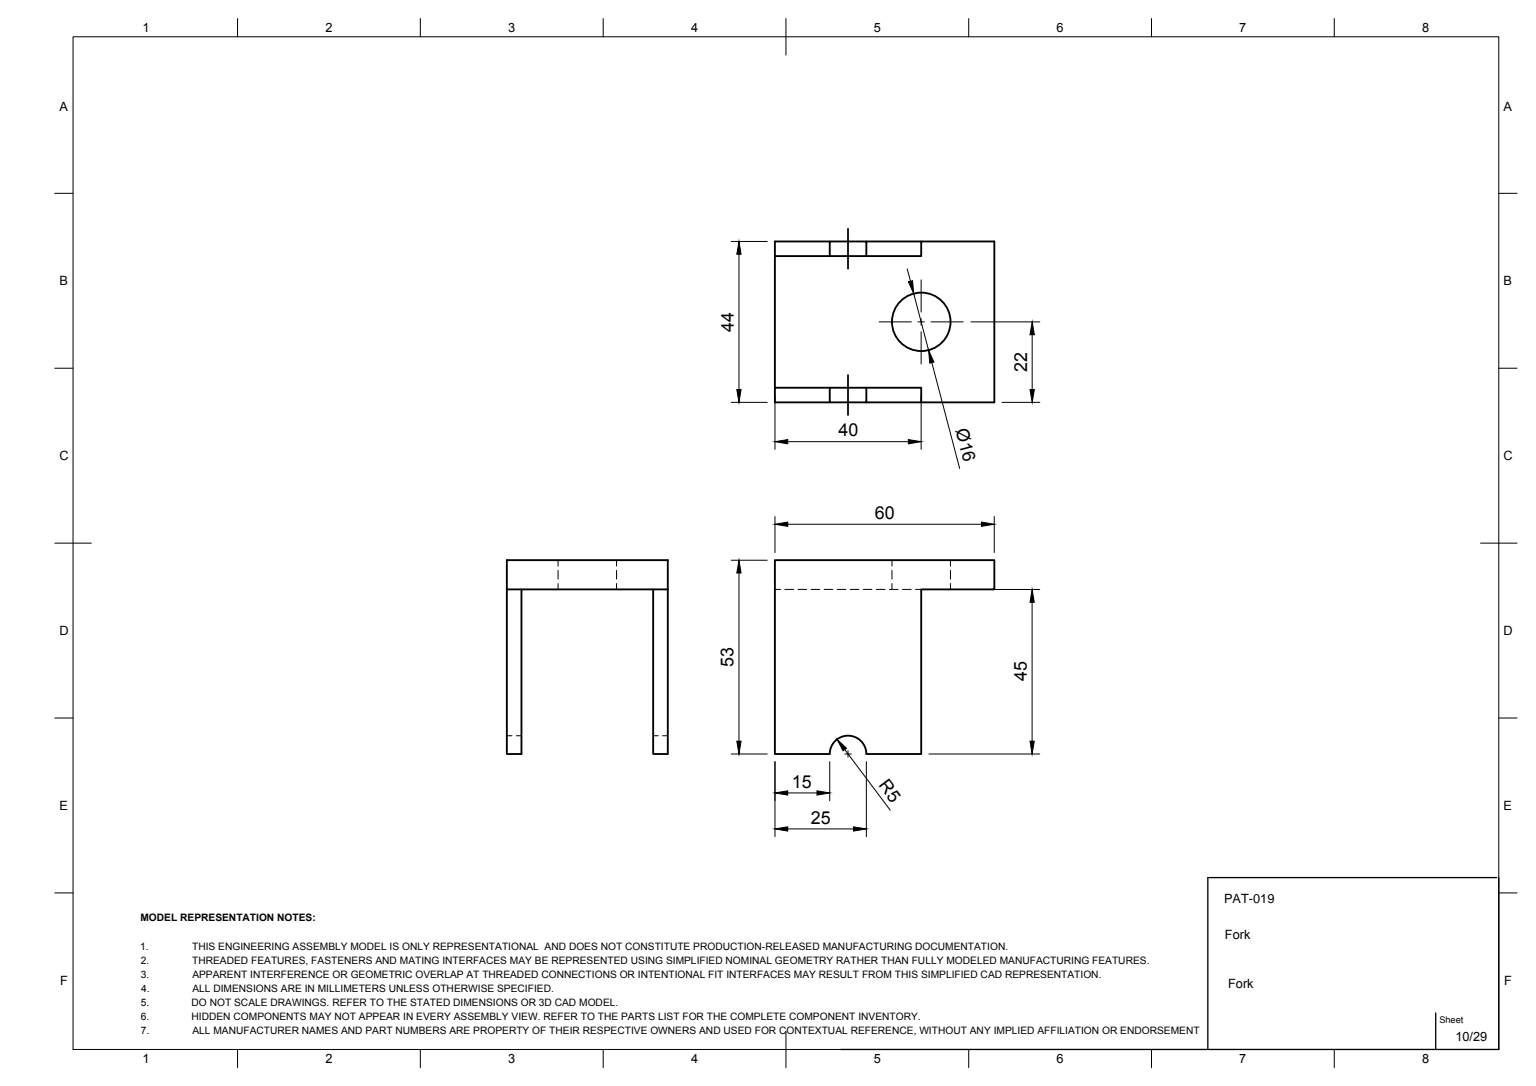
ISO-10303-21;
HEADER;
/* Generated by software containing ST-Developer
 * from STEP Tools, Inc. (www.steptools.com) 
 */

FILE_DESCRIPTION(
/* description */ ('Caster wheel assembly'),
/* implementation_level */ '2;1');

FILE_NAME(
/* name */ 'Fork.step',
/* time_stamp */ '2026-10-28T03:23:56-07:00',
/* author */ (''),
/* organization */ (''),
/* preprocessor_version */ 'ST-DEVELOPER v20.2',
/* originating_system */ 'Autodesk Translation Framework v15.17.0.0',
/* authorisation */ '');

FILE_SCHEMA (('AUTOMOTIVE_DESIGN { 1 0 10303 214 3 1 1 }'));
ENDSEC;

DATA;
#10=MECHANICAL_DESIGN_GEOMETRIC_PRESENTATION_REPRESENTATION('',(#227),#5385);
#183=SHAPE_REPRESENTATION_RELATIONSHIP('SRR','None',#5479,#205);
#205=ADVANCED_BREP_SHAPE_REPRESENTATION('',(#257),#5366);
#227=STYLED_ITEM('',(#5686),#257);
#257=MANIFOLD_SOLID_BREP('Body1',#2654);
#299=FACE_BOUND('',#655,.T.);
#300=FACE_BOUND('',#662,.T.);
#355=PLANE('',#3011);
#356=PLANE('',#3012);
#357=PLANE('',#3013);
#358=PLANE('',#3014);
#359=PLANE('',#3015);
#360=PLANE('',#3016);
#361=PLANE('',#3017);
#362=PLANE('',#3018);
#363=PLANE('',#3019);
#364=PLANE('',#3020);
#365=PLANE('',#3021);
#366=PLANE('',#3022);
#367=PLANE('',#3023);
#368=PLANE('',#3024);
#458=FACE_OUTER_BOUND('',#644,.T.);
#459=FACE_OUTER_BOUND('',#645,.T.);
#460=FACE_OUTER_BOUND('',#646,.T.);
#461=FACE_OUTER_BOUND('',#647,.T.);
#462=FACE_OUTER_BOUND('',#648,.T.);
#463=FACE_OUTER_BOUND('',#649,.T.);
#464=FACE_OUTER_BOUND('',#650,.T.);
#465=FACE_OUTER_BOUND('',#651,.T.);
#466=FACE_OUTER_BOUND('',#652,.T.);
#467=FACE_OUTER_BOUND('',#653,.T.);
#468=FACE_OUTER_BOUND('',#654,.T.);
#469=FACE_OUTER_BOUND('',#656,.T.);
#470=FACE_OUTER_BOUND('',#657,.T.);
#471=FACE_OUTER_BOUND('',#658,.T.);
#472=FACE_OUTER_BOUND('',#659,.T.);
#473=FACE_OUTER_BOUND('',#660,.T.);
#474=FACE_OUTER_BOUND('',#661,.T.);
#644=EDGE_LOOP('',(#1928,#1929,#1930,#1931));
#645=EDGE_LOOP('',(#1932,#1933,#1934,#1935));
#646=EDGE_LOOP('',(#1936,#1937,#1938,#1939));
#647=EDGE_LOOP('',(#1940,#1941,#1942,#1943,#1944,#1945,#1946,#1947));
#648=EDGE_LOOP('',(#1948,#1949,#1950,#1951));
#649=EDGE_LOOP('',(#1952,#1953,#1954,#1955));
#650=EDGE_LOOP('',(#1956,#1957,#1958,#1959,#1960,#1961,#1962,#1963));
#651=EDGE_LOOP('',(#1964,#1965,#1966,#1967));
#652=EDGE_LOOP('',(#1968,#1969,#1970,#1971));
#653=EDGE_LOOP('',(#1972,#1973,#1974,#1975,#1976,#1977));
#654=EDGE_LOOP('',(#1978,#1979,#1980,#1981,#1982,#1983,#1984,#1985));
#655=EDGE_LOOP('',(#1986));
#656=EDGE_LOOP('',(#1987,#1988,#1989,#1990,#1991,#1992,#1993,#1994));
#657=EDGE_LOOP('',(#1995,#1996,#1997,#1998,#1999,#2000));
#658=EDGE_LOOP('',(#2001,#2002,#2003,#2004));
#659=EDGE_LOOP('',(#2005,#2006,#2007,#2008));
#660=EDGE_LOOP('',(#2009,#2010,#2011,#2012));
#661=EDGE_LOOP('',(#2013,#2014,#2015,#2016));
#662=EDGE_LOOP('',(#2017));
#842=LINE('',#4400,#976);
#843=LINE('',#4407,#977);
#844=LINE('',#4410,#978);
#845=LINE('',#4414,#979);
#846=LINE('',#4418,#980);
#847=LINE('',#4422,#981);
#848=LINE('',#4424,#982);
#849=LINE('',#4426,#983);
#850=LINE('',#4428,#984);
#851=LINE('',#4430,#985);
#852=LINE('',#4432,#986);
#853=LINE('',#4433,#987);
#854=LINE('',#4436,#988);
#855=LINE('',#4437,#989);
#856=LINE('',#4440,#990);
#857=LINE('',#4441,#991);
#858=LINE('',#4444,#992);
#859=LINE('',#4446,#993);
#860=LINE('',#4448,#994);
#861=LINE('',#4450,#995);
#862=LINE('',#4452,#996);
#863=LINE('',#4454,#997);
#864=LINE('',#4455,#998);
#865=LINE('',#4458,#999);
#866=LINE('',#4459,#1000);
#867=LINE('',#4462,#1001);
#868=LINE('',#4463,#1002);
#869=LINE('',#4466,#1003);
#870=LINE('',#4467,#1004);
#871=LINE('',#4470,#1005);
#872=LINE('',#4472,#1006);
#873=LINE('',#4473,#1007);
#874=LINE('',#4474,#1008);
#875=LINE('',#4476,#1009);
#876=LINE('',#4477,#1010);
#877=LINE('',#4480,#1011);
#878=LINE('',#4481,#1012);
#879=LINE('',#4483,#1013);
#880=LINE('',#4486,#1014);
#976=VECTOR('',#3499,0.8);
#977=VECTOR('',#3506,1.);
#978=VECTOR('',#3509,1.);
#979=VECTOR('',#3512,1.);
#980=VECTOR('',#3515,1.);
#981=VECTOR('',#3520,1.);
#982=VECTOR('',#3521,1.);
#983=VECTOR('',#3522,1.);
#984=VECTOR('',#3523,1.);
#985=VECTOR('',#3524,1.);
#986=VECTOR('',#3525,1.);
#987=VECTOR('',#3526,1.);
#988=VECTOR('',#3529,1.);
#989=VECTOR('',#3530,1.);
#990=VECTOR('',#3533,1.);
#991=VECTOR('',#3534,1.);
#992=VECTOR('',#3537,1.);
#993=VECTOR('',#3538,1.);
#994=VECTOR('',#3539,1.);
#995=VECTOR('',#3540,1.);
#996=VECTOR('',#3541,1.);
#997=VECTOR('',#3542,1.);
#998=VECTOR('',#3543,1.);
#999=VECTOR('',#3546,1.);
#1000=VECTOR('',#3547,1.);
#1001=VECTOR('',#3550,1.);
#1002=VECTOR('',#3551,1.);
#1003=VECTOR('',#3554,1.);
#1004=VECTOR('',#3555,1.);
#1005=VECTOR('',#3558,1.);
#1006=VECTOR('',#3559,1.);
#1007=VECTOR('',#3560,1.);
#1008=VECTOR('',#3561,1.);
#1009=VECTOR('',#3564,1.);
#1010=VECTOR('',#3565,1.);
#1011=VECTOR('',#3568,1.);
#1012=VECTOR('',#3569,1.);
#1013=VECTOR('',#3572,1.);
#1014=VECTOR('',#3577,1.);
#1105=CIRCLE('',#3003,0.8);
#1106=CIRCLE('',#3004,0.8);
#1107=CIRCLE('',#3006,0.5);
#1108=CIRCLE('',#3007,0.5);
#1109=CIRCLE('',#3009,0.5);
#1110=CIRCLE('',#3010,0.5);
#1284=VERTEX_POINT('',#4397);
#1285=VERTEX_POINT('',#4399);
#1286=VERTEX_POINT('',#4403);
#1287=VERTEX_POINT('',#4404);
#1288=VERTEX_POINT('',#4406);
#1289=VERTEX_POINT('',#4408);
#1290=VERTEX_POINT('',#4412);
#1291=VERTEX_POINT('',#4413);
#1292=VERTEX_POINT('',#4415);
#1293=VERTEX_POINT('',#4417);
#1294=VERTEX_POINT('',#4421);
#1295=VERTEX_POINT('',#4423);
#1296=VERTEX_POINT('',#4425);
#1297=VERTEX_POINT('',#4427);
#1298=VERTEX_POINT('',#4429);
#1299=VERTEX_POINT('',#4431);
#1300=VERTEX_POINT('',#4435);
#1301=VERTEX_POINT('',#4439);
#1302=VERTEX_POINT('',#4443);
#1303=VERTEX_POINT('',#4445);
#1304=VERTEX_POINT('',#4447);
#1305=VERTEX_POINT('',#4449);
#1306=VERTEX_POINT('',#4451);
#1307=VERTEX_POINT('',#4453);
#1308=VERTEX_POINT('',#4457);
#1309=VERTEX_POINT('',#4461);
#1310=VERTEX_POINT('',#4465);
#1311=VERTEX_POINT('',#4469);
#1312=VERTEX_POINT('',#4471);
#1313=VERTEX_POINT('',#4479);
#1532=EDGE_CURVE('',#1284,#1284,#1105,.T.);
#1533=EDGE_CURVE('',#1284,#1285,#842,.T.);
#1534=EDGE_CURVE('',#1285,#1285,#1106,.T.);
#1535=EDGE_CURVE('',#1286,#1287,#1107,.T.);
#1536=EDGE_CURVE('',#1288,#1286,#843,.T.);
#1537=EDGE_CURVE('',#1289,#1288,#1108,.T.);
#1538=EDGE_CURVE('',#1287,#1289,#844,.T.);
#1539=EDGE_CURVE('',#1290,#1291,#845,.T.);
#1540=EDGE_CURVE('',#1292,#1290,#1109,.T.);
#1541=EDGE_CURVE('',#1293,#1292,#846,.T.);
#1542=EDGE_CURVE('',#1291,#1293,#1110,.T.);
#1543=EDGE_CURVE('',#1290,#1294,#847,.T.);
#1544=EDGE_CURVE('',#1294,#1295,#848,.T.);
#1545=EDGE_CURVE('',#1295,#1296,#849,.T.);
#1546=EDGE_CURVE('',#1296,#1297,#850,.T.);
#1547=EDGE_CURVE('',#1298,#1297,#851,.T.);
#1548=EDGE_CURVE('',#1299,#1298,#852,.T.);
#1549=EDGE_CURVE('',#1299,#1292,#853,.T.);
#1550=EDGE_CURVE('',#1300,#1291,#854,.T.);
#1551=EDGE_CURVE('',#1300,#1294,#855,.T.);
#1552=EDGE_CURVE('',#1301,#1299,#856,.T.);
#1553=EDGE_CURVE('',#1293,#1301,#857,.T.);
#1554=EDGE_CURVE('',#1288,#1302,#858,.T.);
#1555=EDGE_CURVE('',#1302,#1303,#859,.T.);
#1556=EDGE_CURVE('',#1304,#1303,#860,.T.);
#1557=EDGE_CURVE('',#1305,#1304,#861,.T.);
#1558=EDGE_CURVE('',#1305,#1306,#862,.T.);
#1559=EDGE_CURVE('',#1306,#1307,#863,.T.);
#1560=EDGE_CURVE('',#1307,#1289,#864,.T.);
#1561=EDGE_CURVE('',#1308,#1286,#865,.T.);
#1562=EDGE_CURVE('',#1302,#1308,#866,.T.);
#1563=EDGE_CURVE('',#1295,#1309,#867,.T.);
#1564=EDGE_CURVE('',#1309,#1300,#868,.T.);
#1565=EDGE_CURVE('',#1301,#1310,#869,.T.);
#1566=EDGE_CURVE('',#1309,#1310,#870,.T.);
#1567=EDGE_CURVE('',#1311,#1310,#871,.T.);
#1568=EDGE_CURVE('',#1311,#1312,#872,.T.);
#1569=EDGE_CURVE('',#1312,#1306,#873,.T.);
#1570=EDGE_CURVE('',#1296,#1305,#874,.T.);
#1571=EDGE_CURVE('',#1303,#1298,#875,.T.);
#1572=EDGE_CURVE('',#1311,#1308,#876,.T.);
#1573=EDGE_CURVE('',#1287,#1313,#877,.T.);
#1574=EDGE_CURVE('',#1313,#1312,#878,.T.);
#1575=EDGE_CURVE('',#1307,#1313,#879,.T.);
#1576=EDGE_CURVE('',#1297,#1304,#880,.T.);
#1928=ORIENTED_EDGE('',*,*,#1532,.F.);
#1929=ORIENTED_EDGE('',*,*,#1533,.T.);
#1930=ORIENTED_EDGE('',*,*,#1534,.F.);
#1931=ORIENTED_EDGE('',*,*,#1533,.F.);
#1932=ORIENTED_EDGE('',*,*,#1535,.F.);
#1933=ORIENTED_EDGE('',*,*,#1536,.F.);
#1934=ORIENTED_EDGE('',*,*,#1537,.F.);
#1935=ORIENTED_EDGE('',*,*,#1538,.F.);
#1936=ORIENTED_EDGE('',*,*,#1539,.F.);
#1937=ORIENTED_EDGE('',*,*,#1540,.F.);
#1938=ORIENTED_EDGE('',*,*,#1541,.F.);
#1939=ORIENTED_EDGE('',*,*,#1542,.F.);
#1940=ORIENTED_EDGE('',*,*,#1540,.T.);
#1941=ORIENTED_EDGE('',*,*,#1543,.T.);
#1942=ORIENTED_EDGE('',*,*,#1544,.T.);
#1943=ORIENTED_EDGE('',*,*,#1545,.T.);
#1944=ORIENTED_EDGE('',*,*,#1546,.T.);
#1945=ORIENTED_EDGE('',*,*,#1547,.F.);
#1946=ORIENTED_EDGE('',*,*,#1548,.F.);
#1947=ORIENTED_EDGE('',*,*,#1549,.T.);
#1948=ORIENTED_EDGE('',*,*,#1539,.T.);
#1949=ORIENTED_EDGE('',*,*,#1550,.F.);
#1950=ORIENTED_EDGE('',*,*,#1551,.T.);
#1951=ORIENTED_EDGE('',*,*,#1543,.F.);
#1952=ORIENTED_EDGE('',*,*,#1541,.T.);
#1953=ORIENTED_EDGE('',*,*,#1549,.F.);
#1954=ORIENTED_EDGE('',*,*,#1552,.F.);
#1955=ORIENTED_EDGE('',*,*,#1553,.F.);
#1956=ORIENTED_EDGE('',*,*,#1537,.T.);
#1957=ORIENTED_EDGE('',*,*,#1554,.T.);
#1958=ORIENTED_EDGE('',*,*,#1555,.T.);
#1959=ORIENTED_EDGE('',*,*,#1556,.F.);
#1960=ORIENTED_EDGE('',*,*,#1557,.F.);
#1961=ORIENTED_EDGE('',*,*,#1558,.T.);
#1962=ORIENTED_EDGE('',*,*,#1559,.T.);
#1963=ORIENTED_EDGE('',*,*,#1560,.T.);
#1964=ORIENTED_EDGE('',*,*,#1536,.T.);
#1965=ORIENTED_EDGE('',*,*,#1561,.F.);
#1966=ORIENTED_EDGE('',*,*,#1562,.F.);
#1967=ORIENTED_EDGE('',*,*,#1554,.F.);
#1968=ORIENTED_EDGE('',*,*,#1563,.F.);
#1969=ORIENTED_EDGE('',*,*,#1544,.F.);
#1970=ORIENTED_EDGE('',*,*,#1551,.F.);
#1971=ORIENTED_EDGE('',*,*,#1564,.F.);
#1972=ORIENTED_EDGE('',*,*,#1542,.T.);
#1973=ORIENTED_EDGE('',*,*,#1553,.T.);
#1974=ORIENTED_EDGE('',*,*,#1565,.T.);
#1975=ORIENTED_EDGE('',*,*,#1566,.F.);
#1976=ORIENTED_EDGE('',*,*,#1564,.T.);
#1977=ORIENTED_EDGE('',*,*,#1550,.T.);
#1978=ORIENTED_EDGE('',*,*,#1563,.T.);
#1979=ORIENTED_EDGE('',*,*,#1566,.T.);
#1980=ORIENTED_EDGE('',*,*,#1567,.F.);
#1981=ORIENTED_EDGE('',*,*,#1568,.T.);
#1982=ORIENTED_EDGE('',*,*,#1569,.T.);
#1983=ORIENTED_EDGE('',*,*,#1558,.F.);
#1984=ORIENTED_EDGE('',*,*,#1570,.F.);
#1985=ORIENTED_EDGE('',*,*,#1545,.F.);
#1986=ORIENTED_EDGE('',*,*,#1532,.T.);
#1987=ORIENTED_EDGE('',*,*,#1548,.T.);
#1988=ORIENTED_EDGE('',*,*,#1571,.F.);
#1989=ORIENTED_EDGE('',*,*,#1555,.F.);
#1990=ORIENTED_EDGE('',*,*,#1562,.T.);
#1991=ORIENTED_EDGE('',*,*,#1572,.F.);
#1992=ORIENTED_EDGE('',*,*,#1567,.T.);
#1993=ORIENTED_EDGE('',*,*,#1565,.F.);
#1994=ORIENTED_EDGE('',*,*,#1552,.T.);
#1995=ORIENTED_EDGE('',*,*,#1535,.T.);
#1996=ORIENTED_EDGE('',*,*,#1573,.T.);
#1997=ORIENTED_EDGE('',*,*,#1574,.T.);
#1998=ORIENTED_EDGE('',*,*,#1568,.F.);
#1999=ORIENTED_EDGE('',*,*,#1572,.T.);
#2000=ORIENTED_EDGE('',*,*,#1561,.T.);
#2001=ORIENTED_EDGE('',*,*,#1569,.F.);
#2002=ORIENTED_EDGE('',*,*,#1574,.F.);
#2003=ORIENTED_EDGE('',*,*,#1575,.F.);
#2004=ORIENTED_EDGE('',*,*,#1559,.F.);
#2005=ORIENTED_EDGE('',*,*,#1538,.T.);
#2006=ORIENTED_EDGE('',*,*,#1560,.F.);
#2007=ORIENTED_EDGE('',*,*,#1575,.T.);
#2008=ORIENTED_EDGE('',*,*,#1573,.F.);
#2009=ORIENTED_EDGE('',*,*,#1570,.T.);
#2010=ORIENTED_EDGE('',*,*,#1557,.T.);
#2011=ORIENTED_EDGE('',*,*,#1576,.F.);
#2012=ORIENTED_EDGE('',*,*,#1546,.F.);
#2013=ORIENTED_EDGE('',*,*,#1576,.T.);
#2014=ORIENTED_EDGE('',*,*,#1556,.T.);
#2015=ORIENTED_EDGE('',*,*,#1571,.T.);
#2016=ORIENTED_EDGE('',*,*,#1547,.T.);
#2017=ORIENTED_EDGE('',*,*,#1534,.T.);
#2441=CYLINDRICAL_SURFACE('',#3002,0.8);
#2442=CYLINDRICAL_SURFACE('',#3005,0.5);
#2443=CYLINDRICAL_SURFACE('',#3008,0.5);
#2518=ADVANCED_FACE('',(#458),#2441,.F.);
#2519=ADVANCED_FACE('',(#459),#2442,.F.);
#2520=ADVANCED_FACE('',(#460),#2443,.F.);
#2521=ADVANCED_FACE('',(#461),#355,.T.);
#2522=ADVANCED_FACE('',(#462),#356,.T.);
#2523=ADVANCED_FACE('',(#463),#357,.T.);
#2524=ADVANCED_FACE('',(#464),#358,.T.);
#2525=ADVANCED_FACE('',(#465),#359,.T.);
#2526=ADVANCED_FACE('',(#466),#360,.T.);
#2527=ADVANCED_FACE('',(#467),#361,.F.);
#2528=ADVANCED_FACE('',(#468,#299),#362,.F.);
#2529=ADVANCED_FACE('',(#469),#363,.T.);
#2530=ADVANCED_FACE('',(#470),#364,.T.);
#2531=ADVANCED_FACE('',(#471),#365,.T.);
#2532=ADVANCED_FACE('',(#472),#366,.T.);
#2533=ADVANCED_FACE('',(#473),#367,.T.);
#2534=ADVANCED_FACE('',(#474,#300),#368,.T.);
#2654=CLOSED_SHELL('',(#2518,#2519,#2520,#2521,#2522,#2523,#2524,#2525,
#2526,#2527,#2528,#2529,#2530,#2531,#2532,#2533,#2534));
#3001=AXIS2_PLACEMENT_3D('',#4395,#3493,#3494);
#3002=AXIS2_PLACEMENT_3D('',#4396,#3495,#3496);
#3003=AXIS2_PLACEMENT_3D('',#4398,#3497,#3498);
#3004=AXIS2_PLACEMENT_3D('',#4401,#3500,#3501);
#3005=AXIS2_PLACEMENT_3D('',#4402,#3502,#3503);
#3006=AXIS2_PLACEMENT_3D('',#4405,#3504,#3505);
#3007=AXIS2_PLACEMENT_3D('',#4409,#3507,#3508);
#3008=AXIS2_PLACEMENT_3D('',#4411,#3510,#3511);
#3009=AXIS2_PLACEMENT_3D('',#4416,#3513,#3514);
#3010=AXIS2_PLACEMENT_3D('',#4419,#3516,#3517);
#3011=AXIS2_PLACEMENT_3D('',#4420,#3518,#3519);
#3012=AXIS2_PLACEMENT_3D('',#4434,#3527,#3528);
#3013=AXIS2_PLACEMENT_3D('',#4438,#3531,#3532);
#3014=AXIS2_PLACEMENT_3D('',#4442,#3535,#3536);
#3015=AXIS2_PLACEMENT_3D('',#4456,#3544,#3545);
#3016=AXIS2_PLACEMENT_3D('',#4460,#3548,#3549);
#3017=AXIS2_PLACEMENT_3D('',#4464,#3552,#3553);
#3018=AXIS2_PLACEMENT_3D('',#4468,#3556,#3557);
#3019=AXIS2_PLACEMENT_3D('',#4475,#3562,#3563);
#3020=AXIS2_PLACEMENT_3D('',#4478,#3566,#3567);
#3021=AXIS2_PLACEMENT_3D('',#4482,#3570,#3571);
#3022=AXIS2_PLACEMENT_3D('',#4484,#3573,#3574);
#3023=AXIS2_PLACEMENT_3D('',#4485,#3575,#3576);
#3024=AXIS2_PLACEMENT_3D('',#4487,#3578,#3579);
#3493=DIRECTION('axis',(0.,0.,1.));
#3494=DIRECTION('refdir',(1.,0.,0.));
#3495=DIRECTION('center_axis',(0.,0.,1.));
#3496=DIRECTION('ref_axis',(1.,0.,0.));
#3497=DIRECTION('center_axis',(0.,0.,1.));
#3498=DIRECTION('ref_axis',(1.,0.,0.));
#3499=DIRECTION('',(0.,0.,1.));
#3500=DIRECTION('center_axis',(0.,0.,-1.));
#3501=DIRECTION('ref_axis',(1.,0.,0.));
#3502=DIRECTION('center_axis',(0.,1.,0.));
#3503=DIRECTION('ref_axis',(1.,0.,0.));
#3504=DIRECTION('center_axis',(0.,-1.,0.));
#3505=DIRECTION('ref_axis',(1.,0.,0.));
#3506=DIRECTION('',(0.,1.,0.));
#3507=DIRECTION('center_axis',(0.,1.,0.));
#3508=DIRECTION('ref_axis',(1.,0.,0.));
#3509=DIRECTION('',(0.,-1.,0.));
#3510=DIRECTION('center_axis',(0.,1.,0.));
#3511=DIRECTION('ref_axis',(1.,0.,0.));
#3512=DIRECTION('',(0.,-1.,0.));
#3513=DIRECTION('center_axis',(0.,-1.,0.));
#3514=DIRECTION('ref_axis',(1.,0.,0.));
#3515=DIRECTION('',(0.,1.,0.));
#3516=DIRECTION('center_axis',(0.,1.,0.));
#3517=DIRECTION('ref_axis',(1.,0.,0.));
#3518=DIRECTION('center_axis',(0.,1.,0.));
#3519=DIRECTION('ref_axis',(-1.,0.,0.));
#3520=DIRECTION('',(-1.,0.,0.));
#3521=DIRECTION('',(0.,0.,1.));
#3522=DIRECTION('',(-1.,0.,0.));
#3523=DIRECTION('',(0.,0.,1.));
#3524=DIRECTION('',(-1.,0.,0.));
#3525=DIRECTION('',(0.,0.,1.));
#3526=DIRECTION('',(-1.,0.,0.));
#3527=DIRECTION('center_axis',(0.,0.,-1.));
#3528=DIRECTION('ref_axis',(-1.,0.,0.));
#3529=DIRECTION('',(1.,0.,0.));
#3530=DIRECTION('',(0.,1.,0.));
#3531=DIRECTION('center_axis',(0.,0.,-1.));
#3532=DIRECTION('ref_axis',(-1.,0.,0.));
#3533=DIRECTION('',(0.,1.,0.));
#3534=DIRECTION('',(1.,0.,0.));
#3535=DIRECTION('center_axis',(0.,-1.,0.));
#3536=DIRECTION('ref_axis',(1.,0.,0.));
#3537=DIRECTION('',(1.,0.,0.));
#3538=DIRECTION('',(0.,0.,1.));
#3539=DIRECTION('',(1.,0.,0.));
#3540=DIRECTION('',(0.,0.,1.));
#3541=DIRECTION('',(1.,0.,0.));
#3542=DIRECTION('',(0.,0.,-1.));
#3543=DIRECTION('',(1.,0.,0.));
#3544=DIRECTION('center_axis',(0.,0.,-1.));
#3545=DIRECTION('ref_axis',(-1.,0.,0.));
#3546=DIRECTION('',(-1.,0.,0.));
#3547=DIRECTION('',(0.,1.,0.));
#3548=DIRECTION('center_axis',(-1.,0.,0.));
#3549=DIRECTION('ref_axis',(0.,0.,1.));
#3550=DIRECTION('',(0.,-1.,0.));
#3551=DIRECTION('',(0.,0.,-1.));
#3552=DIRECTION('center_axis',(0.,1.,0.));
#3553=DIRECTION('ref_axis',(1.,0.,0.));
#3554=DIRECTION('',(0.,0.,1.));
#3555=DIRECTION('',(1.,0.,0.));
#3556=DIRECTION('center_axis',(0.,0.,1.));
#3557=DIRECTION('ref_axis',(1.,0.,0.));
#3558=DIRECTION('',(0.,1.,0.));
#3559=DIRECTION('',(-1.,0.,0.));
#3560=DIRECTION('',(0.,-1.,0.));
#3561=DIRECTION('',(0.,-1.,0.));
#3562=DIRECTION('center_axis',(1.,0.,0.));
#3563=DIRECTION('ref_axis',(0.,1.,0.));
#3564=DIRECTION('',(0.,1.,0.));
#3565=DIRECTION('',(0.,0.,-1.));
#3566=DIRECTION('center_axis',(0.,1.,0.));
#3567=DIRECTION('ref_axis',(0.,0.,1.));
#3568=DIRECTION('',(-1.,0.,0.));
#3569=DIRECTION('',(0.,0.,1.));
#3570=DIRECTION('center_axis',(-1.,0.,0.));
#3571=DIRECTION('ref_axis',(0.,0.,1.));
#3572=DIRECTION('',(0.,1.,0.));
#3573=DIRECTION('center_axis',(0.,0.,-1.));
#3574=DIRECTION('ref_axis',(-1.,0.,0.));
#3575=DIRECTION('center_axis',(-1.,0.,0.));
#3576=DIRECTION('ref_axis',(0.,-1.,0.));
#3577=DIRECTION('',(0.,-1.,0.));
#3578=DIRECTION('center_axis',(0.,0.,1.));
#3579=DIRECTION('ref_axis',(1.,0.,0.));
#4395=CARTESIAN_POINT('',(0.,0.,0.));
#4396=CARTESIAN_POINT('Origin',(-2.,0.,8.4));
#4397=CARTESIAN_POINT('',(-2.8,-9.79717439317883E-17,8.5));
#4398=CARTESIAN_POINT('Origin',(-2.,0.,8.5));
#4399=CARTESIAN_POINT('',(-2.8,9.79717439317883E-17,9.3));
#4400=CARTESIAN_POINT('',(-2.8,-9.79717439317883E-17,8.4));
#4401=CARTESIAN_POINT('Origin',(-2.,0.,9.3));
#4402=CARTESIAN_POINT('Origin',(0.,-2.3,4.));
#4403=CARTESIAN_POINT('',(0.5,-1.8,4.));
#4404=CARTESIAN_POINT('',(-0.5,-1.8,4.));
#4405=CARTESIAN_POINT('Origin',(0.,-1.8,4.));
#4406=CARTESIAN_POINT('',(0.5,-2.2,4.));
#4407=CARTESIAN_POINT('',(0.5,-2.3,4.));
#4408=CARTESIAN_POINT('',(-0.5,-2.2,4.));
#4409=CARTESIAN_POINT('Origin',(0.,-2.2,4.));
#4410=CARTESIAN_POINT('',(-0.5,-2.3,4.));
#4411=CARTESIAN_POINT('Origin',(0.,-2.3,4.));
#4412=CARTESIAN_POINT('',(-0.5,2.2,4.));
#4413=CARTESIAN_POINT('',(-0.5,1.8,4.));
#4414=CARTESIAN_POINT('',(-0.5,-2.3,4.));
#4415=CARTESIAN_POINT('',(0.5,2.2,4.));
#4416=CARTESIAN_POINT('Origin',(0.,2.2,4.));
#4417=CARTESIAN_POINT('',(0.5,1.8,4.));
#4418=CARTESIAN_POINT('',(0.5,-2.3,4.));
#4419=CARTESIAN_POINT('Origin',(0.,1.8,4.));
#4420=CARTESIAN_POINT('Origin',(2.,2.2,8.5));
#4421=CARTESIAN_POINT('',(-2.,2.2,4.));
#4422=CARTESIAN_POINT('',(-2.,2.2,4.));
#4423=CARTESIAN_POINT('',(-2.,2.2,8.5));
#4424=CARTESIAN_POINT('',(-2.,2.2,8.9));
#4425=CARTESIAN_POINT('',(-4.,2.2,8.5));
#4426=CARTESIAN_POINT('',(2.,2.2,8.5));
#4427=CARTESIAN_POINT('',(-4.,2.2,9.3));
#4428=CARTESIAN_POINT('',(-4.,2.2,8.5));
#4429=CARTESIAN_POINT('',(2.,2.2,9.3));
#4430=CARTESIAN_POINT('',(2.,2.2,9.3));
#4431=CARTESIAN_POINT('',(2.,2.2,4.));
#4432=CARTESIAN_POINT('',(2.,2.2,8.5));
#4433=CARTESIAN_POINT('',(-2.,2.2,4.));
#4434=CARTESIAN_POINT('Origin',(2.,1.8,4.));
#4435=CARTESIAN_POINT('',(-2.,1.8,4.));
#4436=CARTESIAN_POINT('',(-2.,1.8,4.));
#4437=CARTESIAN_POINT('',(-2.,1.8,4.));
#4438=CARTESIAN_POINT('Origin',(2.,1.8,4.));
#4439=CARTESIAN_POINT('',(2.,1.8,4.));
#4440=CARTESIAN_POINT('',(2.,1.8,4.));
#4441=CARTESIAN_POINT('',(-2.,1.8,4.));
#4442=CARTESIAN_POINT('Origin',(-4.,-2.2,8.5));
#4443=CARTESIAN_POINT('',(2.,-2.2,4.));
#4444=CARTESIAN_POINT('',(-2.,-2.2,4.));
#4445=CARTESIAN_POINT('',(2.,-2.2,9.3));
#4446=CARTESIAN_POINT('',(2.,-2.2,8.5));
#4447=CARTESIAN_POINT('',(-4.,-2.2,9.3));
#4448=CARTESIAN_POINT('',(-4.,-2.2,9.3));
#4449=CARTESIAN_POINT('',(-4.,-2.2,8.5));
#4450=CARTESIAN_POINT('',(-4.,-2.2,8.5));
#4451=CARTESIAN_POINT('',(-2.,-2.2,8.5));
#4452=CARTESIAN_POINT('',(-4.,-2.2,8.5));
#4453=CARTESIAN_POINT('',(-2.,-2.2,4.));
#4454=CARTESIAN_POINT('',(-2.,-2.2,8.9));
#4455=CARTESIAN_POINT('',(-2.,-2.2,4.));
#4456=CARTESIAN_POINT('Origin',(2.,-2.2,4.));
#4457=CARTESIAN_POINT('',(2.,-1.8,4.));
#4458=CARTESIAN_POINT('',(-2.,-1.8,4.));
#4459=CARTESIAN_POINT('',(2.,-2.2,4.));
#4460=CARTESIAN_POINT('Origin',(-2.,1.8,4.));
#4461=CARTESIAN_POINT('',(-2.,1.8,8.5));
#4462=CARTESIAN_POINT('',(-2.,0.9,8.5));
#4463=CARTESIAN_POINT('',(-2.,1.8,8.9));
#4464=CARTESIAN_POINT('Origin',(0.,1.8,6.45));
#4465=CARTESIAN_POINT('',(2.,1.8,8.5));
#4466=CARTESIAN_POINT('',(2.,1.8,4.));
#4467=CARTESIAN_POINT('',(-0.5,1.8,8.5));
#4468=CARTESIAN_POINT('Origin',(-1.,0.,8.5));
#4469=CARTESIAN_POINT('',(2.,-1.8,8.5));
#4470=CARTESIAN_POINT('',(2.,-2.2,8.5));
#4471=CARTESIAN_POINT('',(-2.,-1.8,8.5));
#4472=CARTESIAN_POINT('',(-0.5,-1.8,8.5));
#4473=CARTESIAN_POINT('',(-2.,-1.1,8.5));
#4474=CARTESIAN_POINT('',(-4.,2.2,8.5));
#4475=CARTESIAN_POINT('Origin',(2.,-2.2,8.5));
#4476=CARTESIAN_POINT('',(2.,-2.2,9.3));
#4477=CARTESIAN_POINT('',(2.,-1.8,4.));
#4478=CARTESIAN_POINT('Origin',(0.,-1.8,6.45));
#4479=CARTESIAN_POINT('',(-2.,-1.8,4.));
#4480=CARTESIAN_POINT('',(-2.,-1.8,4.));
#4481=CARTESIAN_POINT('',(-2.,-1.8,8.9));
#4482=CARTESIAN_POINT('Origin',(-2.,-2.2,4.));
#4483=CARTESIAN_POINT('',(-2.,-2.2,4.));
#4484=CARTESIAN_POINT('Origin',(2.,-2.2,4.));
#4485=CARTESIAN_POINT('Origin',(-4.,2.2,8.5));
#4486=CARTESIAN_POINT('',(-4.,2.2,9.3));
#4487=CARTESIAN_POINT('Origin',(-1.,0.,9.3));
#5338=UNCERTAINTY_MEASURE_WITH_UNIT(LENGTH_MEASURE(0.001),#5386,
'DISTANCE_ACCURACY_VALUE',
'Maximum model space distance between geometric entities at asserted c
onnectivities');
#5357=UNCERTAINTY_MEASURE_WITH_UNIT(LENGTH_MEASURE(0.001),#5386,
'DISTANCE_ACCURACY_VALUE',
'Maximum model space distance between geometric entities at asserted c
onnectivities');
#5366=(
GEOMETRIC_REPRESENTATION_CONTEXT(3)
GLOBAL_UNCERTAINTY_ASSIGNED_CONTEXT((#5338))
GLOBAL_UNIT_ASSIGNED_CONTEXT((#5386,#5388,#5389))
REPRESENTATION_CONTEXT('','3D')
);
#5385=(
GEOMETRIC_REPRESENTATION_CONTEXT(3)
GLOBAL_UNCERTAINTY_ASSIGNED_CONTEXT((#5357))
GLOBAL_UNIT_ASSIGNED_CONTEXT((#5386,#5388,#5389))
REPRESENTATION_CONTEXT('','3D')
);
#5386=(
LENGTH_UNIT()
NAMED_UNIT(*)
SI_UNIT(.CENTI.,.METRE.)
);
#5388=(
NAMED_UNIT(*)
PLANE_ANGLE_UNIT()
SI_UNIT($,.RADIAN.)
);
#5389=(
NAMED_UNIT(*)
SI_UNIT($,.STERADIAN.)
SOLID_ANGLE_UNIT()
);
#5398=SHAPE_DEFINITION_REPRESENTATION(#5430,#5479);
#5430=PRODUCT_DEFINITION_SHAPE('',$,#5507);
#5479=SHAPE_REPRESENTATION('',(#3001),#5366);
#5498=PRODUCT_DEFINITION_CONTEXT('part definition',#5581,'design');
#5507=PRODUCT_DEFINITION('Fork','Fork',#5534,#5498);
#5534=PRODUCT_DEFINITION_FORMATION('',$,#5591);
#5581=APPLICATION_CONTEXT(
'Core Data for Automotive Mechanical Design Process');
#5582=PRODUCT_CONTEXT('part definition',#5581,'mechanical');
#5591=PRODUCT('Fork','Fork','Fork',(#5582));
#5680=COLOUR_RGB('Off White',0.89,0.88,0.83);
#5681=FILL_AREA_STYLE_COLOUR('',#5680);
#5682=FILL_AREA_STYLE('',(#5681));
#5683=SURFACE_STYLE_FILL_AREA(#5682);
#5684=SURFACE_SIDE_STYLE('',(#5683));
#5685=SURFACE_STYLE_USAGE(.BOTH.,#5684);
#5686=PRESENTATION_STYLE_ASSIGNMENT((#5685));
ENDSEC;
END-ISO-10303-21;
